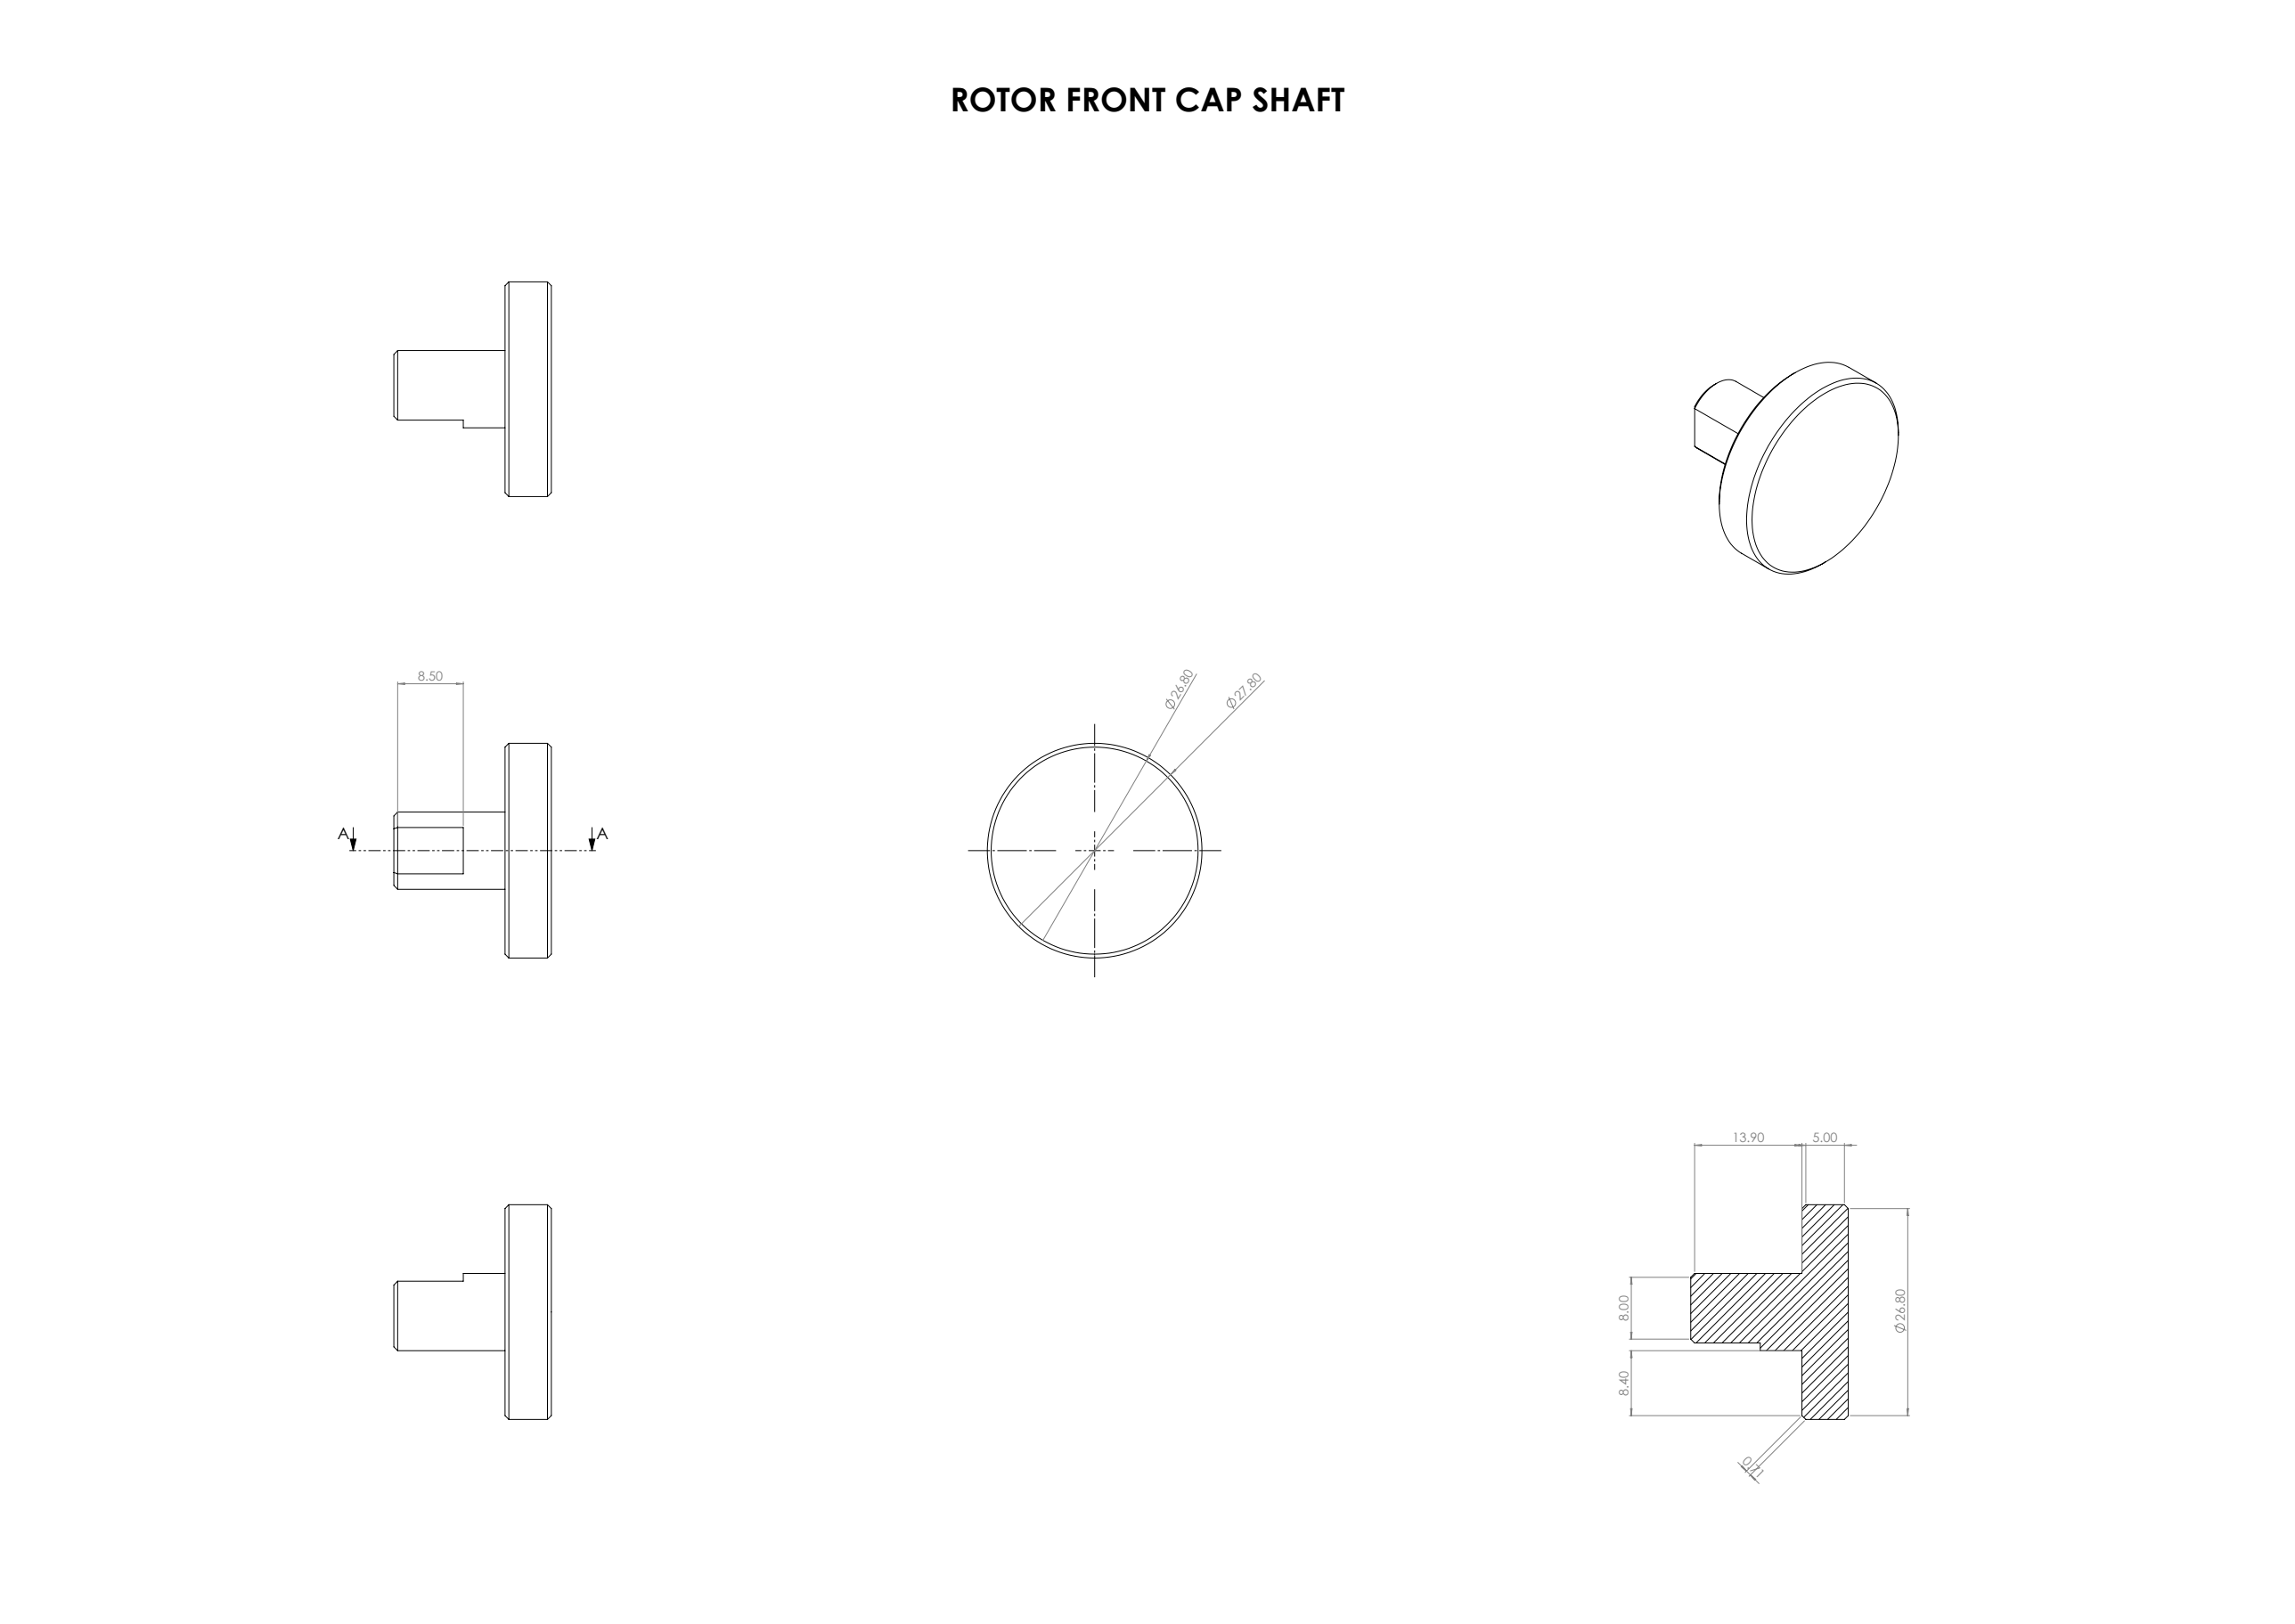
ISO-10303-21;
HEADER;
/* Generated by software containing ST-Developer
 * from STEP Tools, Inc. (www.steptools.com) 
 */

FILE_DESCRIPTION(
/* description */ (''),
/* implementation_level */ '2;1');

FILE_NAME(
/* name */ '04_Rotor_Front_Cap_Shaft.step',
/* time_stamp */ '2026-10-21T01:59:45-07:00',
/* author */ (''),
/* organization */ (''),
/* preprocessor_version */ 'ST-DEVELOPER v20.2',
/* originating_system */ 'Autodesk Translation Framework v15.15.0.0',
/* authorisation */ '');

FILE_SCHEMA (('AUTOMOTIVE_DESIGN { 1 0 10303 214 3 1 1 }'));
ENDSEC;

DATA;
#10=MECHANICAL_DESIGN_GEOMETRIC_PRESENTATION_REPRESENTATION('',(#474),#18281);
#117=(
BOUNDED_CURVE()
B_SPLINE_CURVE(2,(#14471,#14472,#14473),.UNSPECIFIED.,.F.,.F.)
B_SPLINE_CURVE_WITH_KNOTS((3,3),(0.,0.0727628528393549),.UNSPECIFIED.)
CURVE()
GEOMETRIC_REPRESENTATION_ITEM()
RATIONAL_B_SPLINE_CURVE((1.,1.,1.))
REPRESENTATION_ITEM('')
);
#118=(
BOUNDED_CURVE()
B_SPLINE_CURVE(2,(#14477,#14478,#14479),.UNSPECIFIED.,.F.,.F.)
B_SPLINE_CURVE_WITH_KNOTS((3,3),(0.,0.0727628528393549),.UNSPECIFIED.)
CURVE()
GEOMETRIC_REPRESENTATION_ITEM()
RATIONAL_B_SPLINE_CURVE((1.,1.,1.))
REPRESENTATION_ITEM('')
);
#414=CONICAL_SURFACE('',#9675,13.65,0.785398163397449);
#415=CONICAL_SURFACE('',#9683,4.75,0.785398163397446);
#416=CONICAL_SURFACE('',#9695,13.65,0.78539816339745);
#443=SHAPE_REPRESENTATION_RELATIONSHIP('SRR','None',#18345,#456);
#456=ADVANCED_BREP_SHAPE_REPRESENTATION('',(#487),#18274);
#474=STYLED_ITEM('',(#18474),#487);
#487=MANIFOLD_SOLID_BREP('Body1',#9091);
#526=CYLINDRICAL_SURFACE('',#9679,13.9);
#527=CYLINDRICAL_SURFACE('',#9691,5.);
#618=FACE_BOUND('',#1758,.T.);
#737=CIRCLE('',#9676,13.4);
#738=CIRCLE('',#9677,13.9);
#739=CIRCLE('',#9678,13.9);
#740=CIRCLE('',#9680,13.9);
#741=CIRCLE('',#9684,4.5);
#742=CIRCLE('',#9685,5.);
#743=CIRCLE('',#9686,5.);
#744=CIRCLE('',#9689,5.);
#745=CIRCLE('',#9692,5.);
#746=CIRCLE('',#9694,13.4);
#1187=FACE_OUTER_BOUND('',#1748,.T.);
#1188=FACE_OUTER_BOUND('',#1749,.T.);
#1189=FACE_OUTER_BOUND('',#1750,.T.);
#1190=FACE_OUTER_BOUND('',#1751,.T.);
#1191=FACE_OUTER_BOUND('',#1752,.T.);
#1192=FACE_OUTER_BOUND('',#1753,.T.);
#1193=FACE_OUTER_BOUND('',#1754,.T.);
#1194=FACE_OUTER_BOUND('',#1755,.T.);
#1195=FACE_OUTER_BOUND('',#1756,.T.);
#1196=FACE_OUTER_BOUND('',#1757,.T.);
#1197=FACE_OUTER_BOUND('',#1759,.T.);
#1748=EDGE_LOOP('',(#7372,#7373,#7374,#7375,#7376));
#1749=EDGE_LOOP('',(#7377,#7378,#7379,#7380,#7381));
#1750=EDGE_LOOP('',(#7382));
#1751=EDGE_LOOP('',(#7383,#7384,#7385,#7386));
#1752=EDGE_LOOP('',(#7387,#7388,#7389,#7390,#7391));
#1753=EDGE_LOOP('',(#7392,#7393));
#1754=EDGE_LOOP('',(#7394,#7395));
#1755=EDGE_LOOP('',(#7396,#7397,#7398,#7399));
#1756=EDGE_LOOP('',(#7400,#7401,#7402,#7403,#7404,#7405,#7406,#7407));
#1757=EDGE_LOOP('',(#7408));
#1758=EDGE_LOOP('',(#7409));
#1759=EDGE_LOOP('',(#7410,#7411,#7412,#7413));
#2553=LINE('',#14459,#3398);
#2554=LINE('',#14465,#3399);
#2555=LINE('',#14475,#3400);
#2556=LINE('',#14480,#3401);
#2557=LINE('',#14491,#3402);
#2558=LINE('',#14493,#3403);
#2559=LINE('',#14494,#3404);
#2560=LINE('',#14498,#3405);
#2561=LINE('',#14503,#3406);
#3398=VECTOR('',#11457,13.65);
#3399=VECTOR('',#11464,13.9);
#3400=VECTOR('',#11471,10.);
#3401=VECTOR('',#11472,10.);
#3402=VECTOR('',#11487,10.);
#3403=VECTOR('',#11490,10.);
#3404=VECTOR('',#11491,10.);
#3405=VECTOR('',#11496,5.);
#3406=VECTOR('',#11503,13.65);
#4140=VERTEX_POINT('',#14456);
#4141=VERTEX_POINT('',#14458);
#4142=VERTEX_POINT('',#14460);
#4143=VERTEX_POINT('',#14464);
#4144=VERTEX_POINT('',#14469);
#4145=VERTEX_POINT('',#14470);
#4146=VERTEX_POINT('',#14474);
#4147=VERTEX_POINT('',#14476);
#4148=VERTEX_POINT('',#14483);
#4149=VERTEX_POINT('',#14488);
#4150=VERTEX_POINT('',#14489);
#4151=VERTEX_POINT('',#14496);
#4152=VERTEX_POINT('',#14500);
#5258=EDGE_CURVE('',#4140,#4140,#737,.T.);
#5259=EDGE_CURVE('',#4140,#4141,#2553,.T.);
#5260=EDGE_CURVE('',#4141,#4142,#738,.T.);
#5261=EDGE_CURVE('',#4142,#4141,#739,.T.);
#5262=EDGE_CURVE('',#4142,#4143,#2554,.T.);
#5263=EDGE_CURVE('',#4143,#4143,#740,.T.);
#5264=EDGE_CURVE('',#4144,#4145,#117,.T.);
#5265=EDGE_CURVE('',#4145,#4146,#2555,.T.);
#5266=EDGE_CURVE('',#4146,#4147,#118,.T.);
#5267=EDGE_CURVE('',#4147,#4144,#2556,.T.);
#5268=EDGE_CURVE('',#4146,#4145,#741,.T.);
#5269=EDGE_CURVE('',#4148,#4144,#742,.T.);
#5270=EDGE_CURVE('',#4147,#4148,#743,.T.);
#5271=EDGE_CURVE('',#4149,#4150,#744,.T.);
#5272=EDGE_CURVE('',#4150,#4149,#2557,.T.);
#5273=EDGE_CURVE('',#4150,#4147,#2558,.T.);
#5274=EDGE_CURVE('',#4144,#4149,#2559,.T.);
#5275=EDGE_CURVE('',#4151,#4151,#745,.T.);
#5276=EDGE_CURVE('',#4151,#4148,#2560,.T.);
#5277=EDGE_CURVE('',#4152,#4152,#746,.T.);
#5278=EDGE_CURVE('',#4143,#4152,#2561,.T.);
#7372=ORIENTED_EDGE('',*,*,#5258,.T.);
#7373=ORIENTED_EDGE('',*,*,#5259,.T.);
#7374=ORIENTED_EDGE('',*,*,#5260,.T.);
#7375=ORIENTED_EDGE('',*,*,#5261,.T.);
#7376=ORIENTED_EDGE('',*,*,#5259,.F.);
#7377=ORIENTED_EDGE('',*,*,#5260,.F.);
#7378=ORIENTED_EDGE('',*,*,#5261,.F.);
#7379=ORIENTED_EDGE('',*,*,#5262,.T.);
#7380=ORIENTED_EDGE('',*,*,#5263,.T.);
#7381=ORIENTED_EDGE('',*,*,#5262,.F.);
#7382=ORIENTED_EDGE('',*,*,#5258,.F.);
#7383=ORIENTED_EDGE('',*,*,#5264,.T.);
#7384=ORIENTED_EDGE('',*,*,#5265,.T.);
#7385=ORIENTED_EDGE('',*,*,#5266,.T.);
#7386=ORIENTED_EDGE('',*,*,#5267,.T.);
#7387=ORIENTED_EDGE('',*,*,#5266,.F.);
#7388=ORIENTED_EDGE('',*,*,#5268,.T.);
#7389=ORIENTED_EDGE('',*,*,#5264,.F.);
#7390=ORIENTED_EDGE('',*,*,#5269,.F.);
#7391=ORIENTED_EDGE('',*,*,#5270,.F.);
#7392=ORIENTED_EDGE('',*,*,#5265,.F.);
#7393=ORIENTED_EDGE('',*,*,#5268,.F.);
#7394=ORIENTED_EDGE('',*,*,#5271,.F.);
#7395=ORIENTED_EDGE('',*,*,#5272,.F.);
#7396=ORIENTED_EDGE('',*,*,#5267,.F.);
#7397=ORIENTED_EDGE('',*,*,#5273,.F.);
#7398=ORIENTED_EDGE('',*,*,#5272,.T.);
#7399=ORIENTED_EDGE('',*,*,#5274,.F.);
#7400=ORIENTED_EDGE('',*,*,#5275,.F.);
#7401=ORIENTED_EDGE('',*,*,#5276,.T.);
#7402=ORIENTED_EDGE('',*,*,#5269,.T.);
#7403=ORIENTED_EDGE('',*,*,#5274,.T.);
#7404=ORIENTED_EDGE('',*,*,#5271,.T.);
#7405=ORIENTED_EDGE('',*,*,#5273,.T.);
#7406=ORIENTED_EDGE('',*,*,#5270,.T.);
#7407=ORIENTED_EDGE('',*,*,#5276,.F.);
#7408=ORIENTED_EDGE('',*,*,#5277,.F.);
#7409=ORIENTED_EDGE('',*,*,#5275,.T.);
#7410=ORIENTED_EDGE('',*,*,#5263,.F.);
#7411=ORIENTED_EDGE('',*,*,#5278,.T.);
#7412=ORIENTED_EDGE('',*,*,#5277,.T.);
#7413=ORIENTED_EDGE('',*,*,#5278,.F.);
#8467=PLANE('',#9681);
#8468=PLANE('',#9682);
#8469=PLANE('',#9687);
#8470=PLANE('',#9688);
#8471=PLANE('',#9690);
#8472=PLANE('',#9693);
#8908=ADVANCED_FACE('',(#1187),#414,.T.);
#8909=ADVANCED_FACE('',(#1188),#526,.T.);
#8910=ADVANCED_FACE('',(#1189),#8467,.T.);
#8911=ADVANCED_FACE('',(#1190),#8468,.T.);
#8912=ADVANCED_FACE('',(#1191),#415,.T.);
#8913=ADVANCED_FACE('',(#1192),#8469,.T.);
#8914=ADVANCED_FACE('',(#1193),#8470,.F.);
#8915=ADVANCED_FACE('',(#1194),#8471,.F.);
#8916=ADVANCED_FACE('',(#1195),#527,.T.);
#8917=ADVANCED_FACE('',(#1196,#618),#8472,.T.);
#8918=ADVANCED_FACE('',(#1197),#416,.T.);
#9091=CLOSED_SHELL('',(#8908,#8909,#8910,#8911,#8912,#8913,#8914,#8915,
#8916,#8917,#8918));
#9674=AXIS2_PLACEMENT_3D('',#14454,#11451,#11452);
#9675=AXIS2_PLACEMENT_3D('',#14455,#11453,#11454);
#9676=AXIS2_PLACEMENT_3D('',#14457,#11455,#11456);
#9677=AXIS2_PLACEMENT_3D('',#14461,#11458,#11459);
#9678=AXIS2_PLACEMENT_3D('',#14462,#11460,#11461);
#9679=AXIS2_PLACEMENT_3D('',#14463,#11462,#11463);
#9680=AXIS2_PLACEMENT_3D('',#14466,#11465,#11466);
#9681=AXIS2_PLACEMENT_3D('',#14467,#11467,#11468);
#9682=AXIS2_PLACEMENT_3D('',#14468,#11469,#11470);
#9683=AXIS2_PLACEMENT_3D('',#14481,#11473,#11474);
#9684=AXIS2_PLACEMENT_3D('',#14482,#11475,#11476);
#9685=AXIS2_PLACEMENT_3D('',#14484,#11477,#11478);
#9686=AXIS2_PLACEMENT_3D('',#14485,#11479,#11480);
#9687=AXIS2_PLACEMENT_3D('',#14486,#11481,#11482);
#9688=AXIS2_PLACEMENT_3D('',#14487,#11483,#11484);
#9689=AXIS2_PLACEMENT_3D('',#14490,#11485,#11486);
#9690=AXIS2_PLACEMENT_3D('',#14492,#11488,#11489);
#9691=AXIS2_PLACEMENT_3D('',#14495,#11492,#11493);
#9692=AXIS2_PLACEMENT_3D('',#14497,#11494,#11495);
#9693=AXIS2_PLACEMENT_3D('',#14499,#11497,#11498);
#9694=AXIS2_PLACEMENT_3D('',#14501,#11499,#11500);
#9695=AXIS2_PLACEMENT_3D('',#14502,#11501,#11502);
#11451=DIRECTION('axis',(0.,0.,1.));
#11452=DIRECTION('refdir',(1.,0.,0.));
#11453=DIRECTION('center_axis',(-1.,0.,0.));
#11454=DIRECTION('ref_axis',(0.,-1.,0.));
#11455=DIRECTION('center_axis',(-1.,0.,0.));
#11456=DIRECTION('ref_axis',(0.,-1.,0.));
#11457=DIRECTION('',(-0.707106781186547,0.707106781186548,8.65956056235494E-17));
#11458=DIRECTION('center_axis',(1.,0.,0.));
#11459=DIRECTION('ref_axis',(0.,-1.,0.));
#11460=DIRECTION('center_axis',(1.,0.,0.));
#11461=DIRECTION('ref_axis',(0.,-1.,0.));
#11462=DIRECTION('center_axis',(1.,0.,0.));
#11463=DIRECTION('ref_axis',(0.,1.,0.));
#11464=DIRECTION('',(-1.,0.,0.));
#11465=DIRECTION('center_axis',(1.,0.,0.));
#11466=DIRECTION('ref_axis',(0.,0.,-1.));
#11467=DIRECTION('center_axis',(1.,0.,0.));
#11468=DIRECTION('ref_axis',(0.,0.,-1.));
#11469=DIRECTION('center_axis',(-0.707106781186549,0.,0.707106781186546));
#11470=DIRECTION('ref_axis',(0.707106781186546,0.,0.707106781186549));
#11471=DIRECTION('',(0.,-1.,0.));
#11472=DIRECTION('',(0.,1.,0.));
#11473=DIRECTION('center_axis',(1.,0.,0.));
#11474=DIRECTION('ref_axis',(0.,-1.83697019872103E-16,-1.));
#11475=DIRECTION('center_axis',(1.,0.,0.));
#11476=DIRECTION('ref_axis',(0.,0.,-1.));
#11477=DIRECTION('center_axis',(1.,0.,0.));
#11478=DIRECTION('ref_axis',(0.,0.,-1.));
#11479=DIRECTION('center_axis',(1.,0.,0.));
#11480=DIRECTION('ref_axis',(0.,0.,-1.));
#11481=DIRECTION('center_axis',(-1.,0.,0.));
#11482=DIRECTION('ref_axis',(0.,0.,1.));
#11483=DIRECTION('center_axis',(1.,0.,0.));
#11484=DIRECTION('ref_axis',(0.,0.,-1.));
#11485=DIRECTION('center_axis',(1.,0.,0.));
#11486=DIRECTION('ref_axis',(0.,1.,0.));
#11487=DIRECTION('',(0.,1.,0.));
#11488=DIRECTION('center_axis',(0.,0.,-1.));
#11489=DIRECTION('ref_axis',(0.,1.,0.));
#11490=DIRECTION('',(-1.,0.,0.));
#11491=DIRECTION('',(1.,0.,0.));
#11492=DIRECTION('center_axis',(1.,0.,0.));
#11493=DIRECTION('ref_axis',(0.,1.,0.));
#11494=DIRECTION('center_axis',(1.,0.,0.));
#11495=DIRECTION('ref_axis',(0.,0.,-1.));
#11496=DIRECTION('',(-1.,0.,0.));
#11497=DIRECTION('center_axis',(-1.,0.,0.));
#11498=DIRECTION('ref_axis',(0.,0.,1.));
#11499=DIRECTION('center_axis',(1.,0.,0.));
#11500=DIRECTION('ref_axis',(0.,0.,-1.));
#11501=DIRECTION('center_axis',(1.,0.,0.));
#11502=DIRECTION('ref_axis',(0.,1.,0.));
#11503=DIRECTION('',(-0.707106781186547,0.707106781186548,8.65956056235494E-17));
#14454=CARTESIAN_POINT('',(0.,0.,0.));
#14455=CARTESIAN_POINT('Origin',(-0.25,0.,0.));
#14456=CARTESIAN_POINT('',(0.,13.4,-1.64102671085745E-15));
#14457=CARTESIAN_POINT('Origin',(0.,0.,0.));
#14458=CARTESIAN_POINT('',(-0.5,13.9,1.70225905081482E-15));
#14459=CARTESIAN_POINT('',(-0.25,13.65,1.67164288083614E-15));
#14460=CARTESIAN_POINT('',(-0.5,-13.9,-1.70225905081482E-15));
#14461=CARTESIAN_POINT('Origin',(-0.5,0.,0.));
#14462=CARTESIAN_POINT('Origin',(-0.5,0.,0.));
#14463=CARTESIAN_POINT('Origin',(-2.75,0.,0.));
#14464=CARTESIAN_POINT('',(-5.5,-13.9,-1.70225905081482E-15));
#14465=CARTESIAN_POINT('',(-2.75,-13.9,-1.70225905081482E-15));
#14466=CARTESIAN_POINT('Origin',(-5.5,0.,0.));
#14467=CARTESIAN_POINT('Origin',(0.,0.,0.));
#14468=CARTESIAN_POINT('Origin',(-20.15,-0.75,3.75));
#14469=CARTESIAN_POINT('',(-19.9,3.,4.));
#14470=CARTESIAN_POINT('',(-20.4,2.82842712474619,3.5));
#14471=CARTESIAN_POINT('Ctrl Pts',(-19.9,2.99999999999999,4.00000000000001));
#14472=CARTESIAN_POINT('Ctrl Pts',(-20.157359312881,2.914213562373,3.74264068711902));
#14473=CARTESIAN_POINT('Ctrl Pts',(-20.4,2.82842712474619,3.5));
#14474=CARTESIAN_POINT('',(-20.4,-2.82842712474619,3.5));
#14475=CARTESIAN_POINT('',(-20.4,-0.75,3.5));
#14476=CARTESIAN_POINT('',(-19.9,-3.,4.));
#14477=CARTESIAN_POINT('Ctrl Pts',(-20.4,-2.82842712474619,3.5));
#14478=CARTESIAN_POINT('Ctrl Pts',(-20.157359312881,-2.914213562373,3.74264068711902));
#14479=CARTESIAN_POINT('Ctrl Pts',(-19.9,-2.99999999999999,4.00000000000001));
#14480=CARTESIAN_POINT('',(-19.9,-0.75,4.));
#14481=CARTESIAN_POINT('Origin',(-20.15,0.,0.));
#14482=CARTESIAN_POINT('Origin',(-20.4,0.,0.));
#14483=CARTESIAN_POINT('',(-19.9,-5.,-6.12323399573677E-16));
#14484=CARTESIAN_POINT('Origin',(-19.9,0.,0.));
#14485=CARTESIAN_POINT('Origin',(-19.9,0.,0.));
#14486=CARTESIAN_POINT('Origin',(-20.4,4.5,0.));
#14487=CARTESIAN_POINT('Origin',(-11.4,0.,5.));
#14488=CARTESIAN_POINT('',(-11.4,3.,4.));
#14489=CARTESIAN_POINT('',(-11.4,-3.,4.));
#14490=CARTESIAN_POINT('Origin',(-11.4,0.,0.));
#14491=CARTESIAN_POINT('',(-11.4,-6.,4.));
#14492=CARTESIAN_POINT('Origin',(-20.4,-6.,4.));
#14493=CARTESIAN_POINT('',(-12.95,-3.,4.));
#14494=CARTESIAN_POINT('',(-12.95,3.,4.));
#14495=CARTESIAN_POINT('Origin',(-12.95,0.,0.));
#14496=CARTESIAN_POINT('',(-6.,-5.,-6.12323399573677E-16));
#14497=CARTESIAN_POINT('Origin',(-6.,0.,0.));
#14498=CARTESIAN_POINT('',(-12.95,-5.,-6.12323399573677E-16));
#14499=CARTESIAN_POINT('Origin',(-6.,13.4,0.));
#14500=CARTESIAN_POINT('',(-6.,-13.4,-1.64102671085745E-15));
#14501=CARTESIAN_POINT('Origin',(-6.,0.,0.));
#14502=CARTESIAN_POINT('Origin',(-5.75,0.,0.));
#14503=CARTESIAN_POINT('',(-5.75,-13.65,-1.67164288083614E-15));
#18259=UNCERTAINTY_MEASURE_WITH_UNIT(LENGTH_MEASURE(0.01),#18282,
'DISTANCE_ACCURACY_VALUE',
'Maximum model space distance between geometric entities at asserted c
onnectivities');
#18266=UNCERTAINTY_MEASURE_WITH_UNIT(LENGTH_MEASURE(0.01),#18282,
'DISTANCE_ACCURACY_VALUE',
'Maximum model space distance between geometric entities at asserted c
onnectivities');
#18274=(
GEOMETRIC_REPRESENTATION_CONTEXT(3)
GLOBAL_UNCERTAINTY_ASSIGNED_CONTEXT((#18259))
GLOBAL_UNIT_ASSIGNED_CONTEXT((#18282,#18284,#18285))
REPRESENTATION_CONTEXT('','3D')
);
#18281=(
GEOMETRIC_REPRESENTATION_CONTEXT(3)
GLOBAL_UNCERTAINTY_ASSIGNED_CONTEXT((#18266))
GLOBAL_UNIT_ASSIGNED_CONTEXT((#18282,#18284,#18285))
REPRESENTATION_CONTEXT('','3D')
);
#18282=(
LENGTH_UNIT()
NAMED_UNIT(*)
SI_UNIT(.MILLI.,.METRE.)
);
#18284=(
NAMED_UNIT(*)
PLANE_ANGLE_UNIT()
SI_UNIT($,.RADIAN.)
);
#18285=(
NAMED_UNIT(*)
SI_UNIT($,.STERADIAN.)
SOLID_ANGLE_UNIT()
);
#18293=SHAPE_DEFINITION_REPRESENTATION(#18307,#18345);
#18307=PRODUCT_DEFINITION_SHAPE('',$,#18360);
#18345=SHAPE_REPRESENTATION('',(#9674),#18274);
#18352=PRODUCT_DEFINITION_CONTEXT('part definition',#18396,'design');
#18360=PRODUCT_DEFINITION('2026-10-20-13-03-18-510',
'04_Rotor_Front_Cap_Shaft',#18374,#18352);
#18374=PRODUCT_DEFINITION_FORMATION('',$,#18405);
#18396=APPLICATION_CONTEXT(
'Core Data for Automotive Mechanical Design Process');
#18397=PRODUCT_CONTEXT('part definition',#18396,'mechanical');
#18405=PRODUCT('2026-10-20-13-03-18-510','04_Rotor_Front_Cap_Shaft',$,(#18397));
#18468=COLOUR_RGB('Grey',0.48,0.52,0.57);
#18469=FILL_AREA_STYLE_COLOUR('',#18468);
#18470=FILL_AREA_STYLE('',(#18469));
#18471=SURFACE_STYLE_FILL_AREA(#18470);
#18472=SURFACE_SIDE_STYLE('',(#18471));
#18473=SURFACE_STYLE_USAGE(.BOTH.,#18472);
#18474=PRESENTATION_STYLE_ASSIGNMENT((#18473));
ENDSEC;
END-ISO-10303-21;
